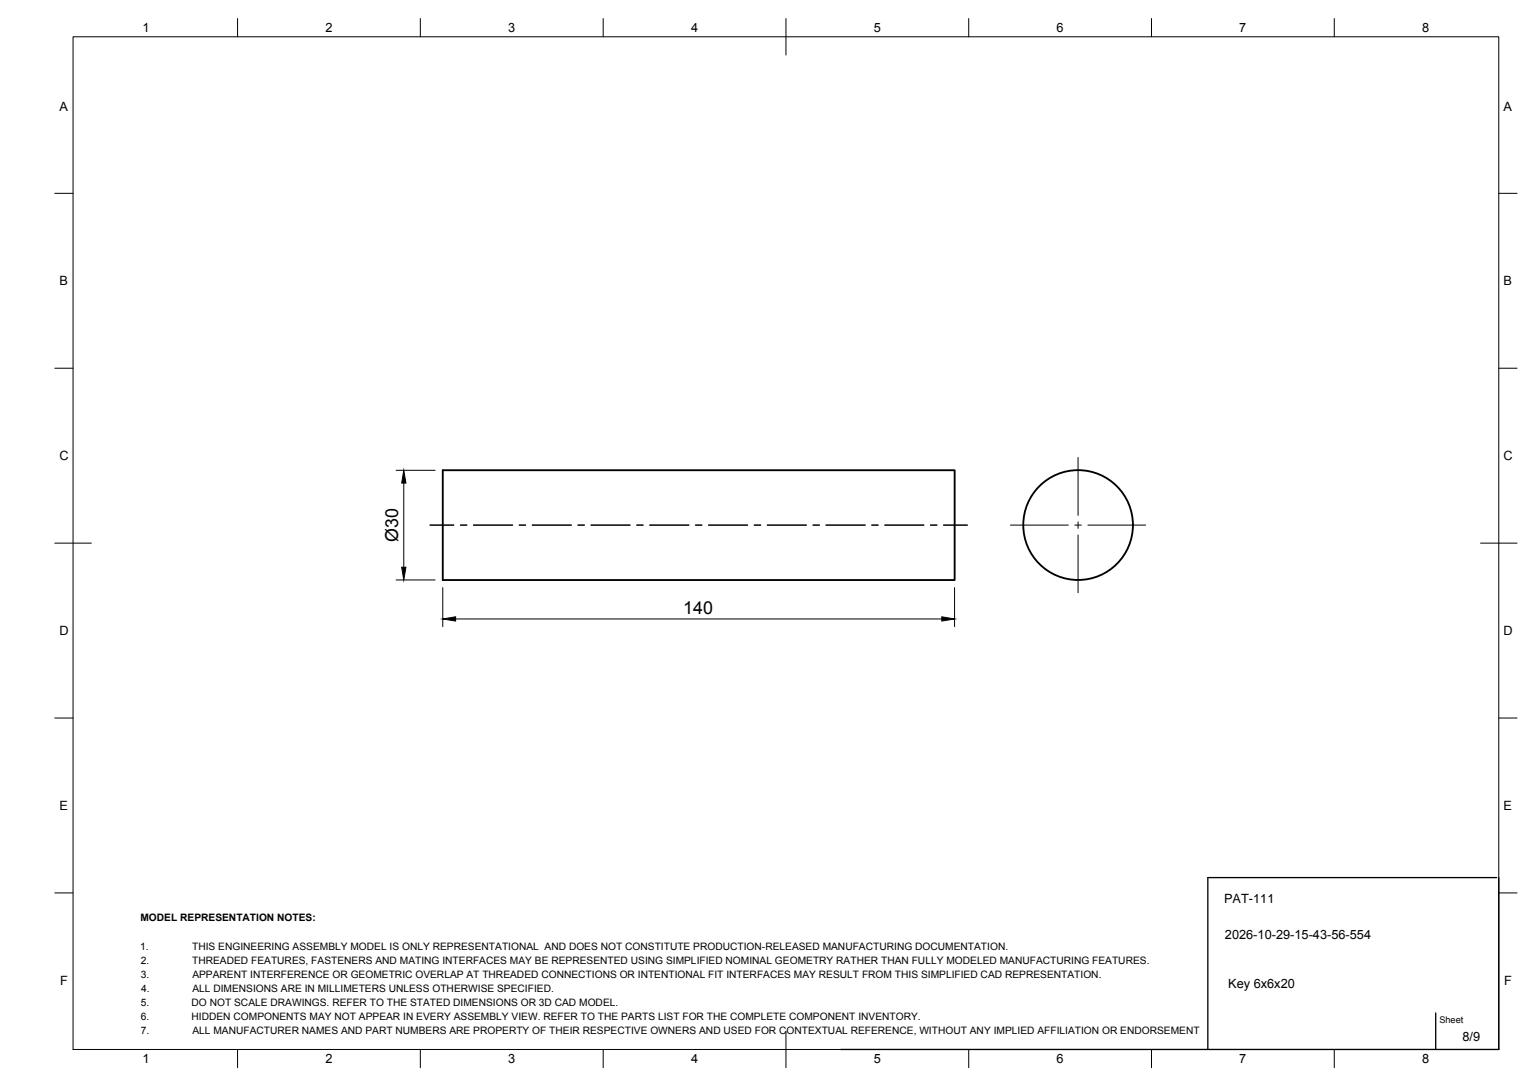
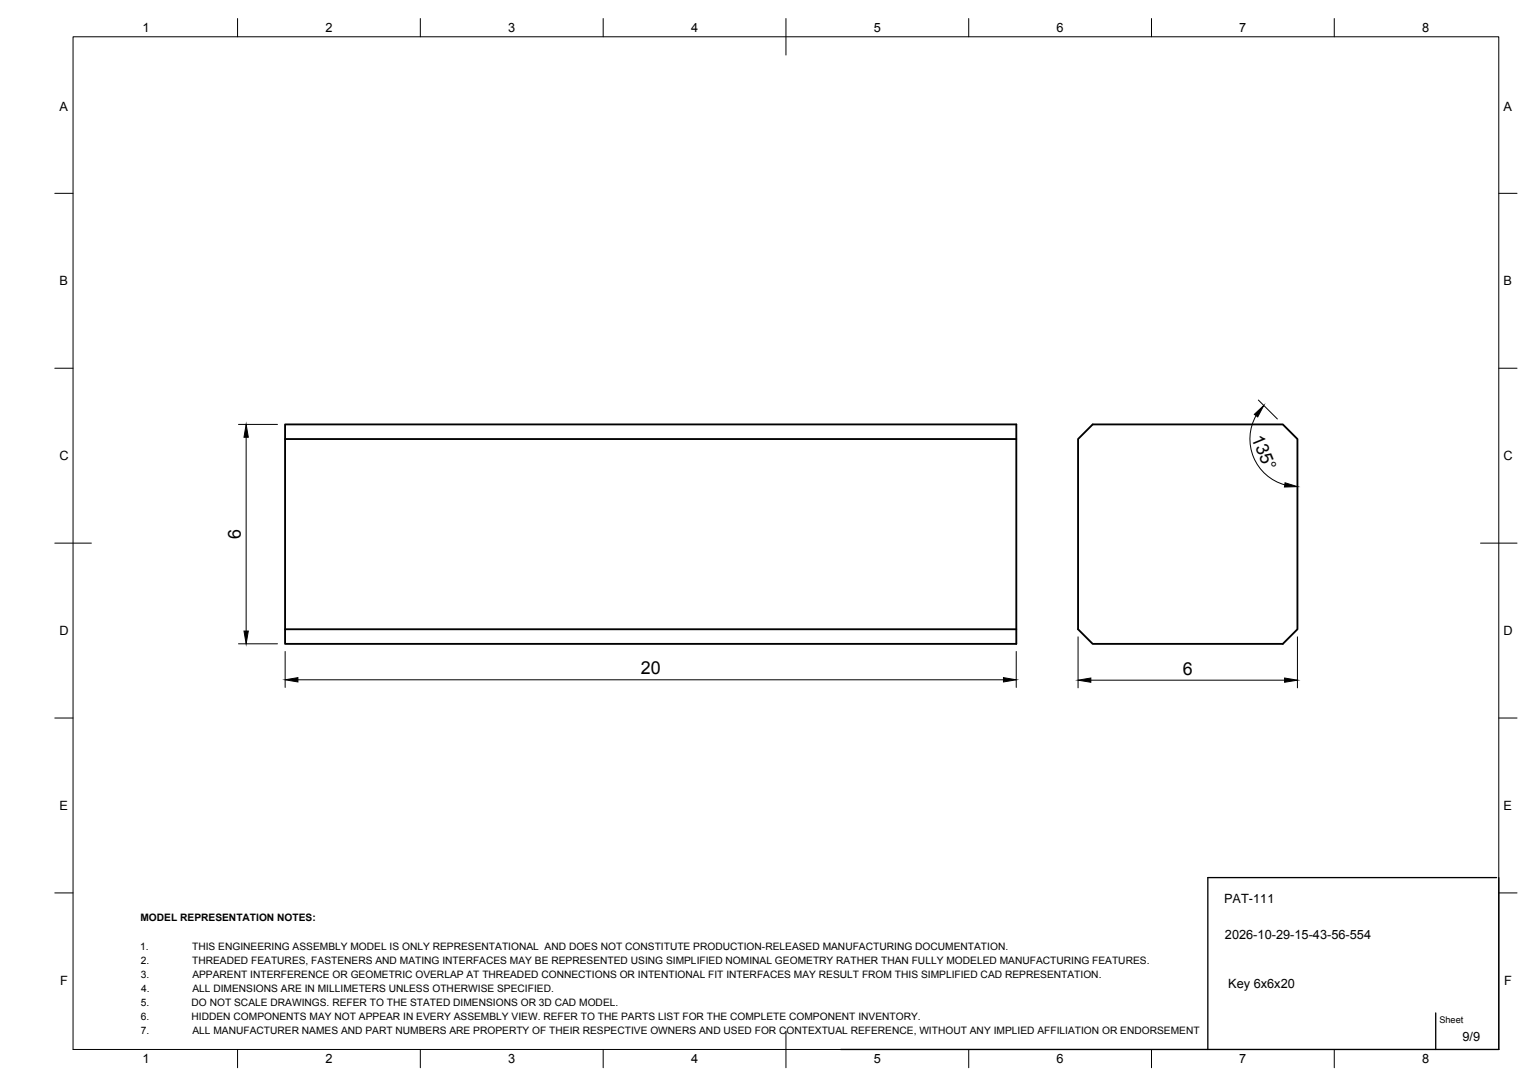
ISO-10303-21;
HEADER;
/* Generated by software containing ST-Developer
 * from STEP Tools, Inc. (www.steptools.com) 
 */

FILE_DESCRIPTION(
/* description */ ('Grid plate located blocks and clamp'),
/* implementation_level */ '2;1');

FILE_NAME(
/* name */ 'Key 6x6x20.step',
/* time_stamp */ '2026-10-29T15:43:47-07:00',
/* author */ (''),
/* organization */ (''),
/* preprocessor_version */ 'ST-DEVELOPER v20.2',
/* originating_system */ 'Autodesk Translation Framework v15.17.0.0',
/* authorisation */ '');

FILE_SCHEMA (('AUTOMOTIVE_DESIGN { 1 0 10303 214 3 1 1 }'));
ENDSEC;

DATA;
#10=MECHANICAL_DESIGN_GEOMETRIC_PRESENTATION_REPRESENTATION('',(#167),#5702);
#143=SHAPE_REPRESENTATION_RELATIONSHIP('SRR','None',#5761,#155);
#155=ADVANCED_BREP_SHAPE_REPRESENTATION('',(#181),#5691);
#167=STYLED_ITEM('',(#5897),#181);
#181=MANIFOLD_SOLID_BREP('Body1',#3262);
#498=FACE_OUTER_BOUND('',#733,.T.);
#499=FACE_OUTER_BOUND('',#734,.T.);
#500=FACE_OUTER_BOUND('',#735,.T.);
#501=FACE_OUTER_BOUND('',#736,.T.);
#502=FACE_OUTER_BOUND('',#737,.T.);
#503=FACE_OUTER_BOUND('',#738,.T.);
#504=FACE_OUTER_BOUND('',#739,.T.);
#505=FACE_OUTER_BOUND('',#740,.T.);
#506=FACE_OUTER_BOUND('',#741,.T.);
#507=FACE_OUTER_BOUND('',#742,.T.);
#733=EDGE_LOOP('',(#2354,#2355,#2356,#2357,#2358,#2359,#2360,#2361));
#734=EDGE_LOOP('',(#2362,#2363,#2364,#2365));
#735=EDGE_LOOP('',(#2366,#2367,#2368,#2369));
#736=EDGE_LOOP('',(#2370,#2371,#2372,#2373));
#737=EDGE_LOOP('',(#2374,#2375,#2376,#2377));
#738=EDGE_LOOP('',(#2378,#2379,#2380,#2381,#2382,#2383,#2384,#2385));
#739=EDGE_LOOP('',(#2386,#2387,#2388,#2389));
#740=EDGE_LOOP('',(#2390,#2391,#2392,#2393));
#741=EDGE_LOOP('',(#2394,#2395,#2396,#2397));
#742=EDGE_LOOP('',(#2398,#2399,#2400,#2401));
#960=LINE('',#4974,#1233);
#961=LINE('',#4976,#1234);
#962=LINE('',#4978,#1235);
#963=LINE('',#4980,#1236);
#964=LINE('',#4982,#1237);
#965=LINE('',#4984,#1238);
#966=LINE('',#4986,#1239);
#967=LINE('',#4987,#1240);
#968=LINE('',#4990,#1241);
#969=LINE('',#4992,#1242);
#970=LINE('',#4993,#1243);
#971=LINE('',#4996,#1244);
#972=LINE('',#4997,#1245);
#973=LINE('',#5000,#1246);
#974=LINE('',#5001,#1247);
#975=LINE('',#5004,#1248);
#976=LINE('',#5005,#1249);
#977=LINE('',#5009,#1250);
#978=LINE('',#5010,#1251);
#979=LINE('',#5012,#1252);
#980=LINE('',#5013,#1253);
#981=LINE('',#5015,#1254);
#982=LINE('',#5017,#1255);
#983=LINE('',#5019,#1256);
#1233=VECTOR('',#4014,1.);
#1234=VECTOR('',#4015,1.);
#1235=VECTOR('',#4016,1.);
#1236=VECTOR('',#4017,1.);
#1237=VECTOR('',#4018,1.);
#1238=VECTOR('',#4019,1.);
#1239=VECTOR('',#4020,1.);
#1240=VECTOR('',#4021,1.);
#1241=VECTOR('',#4024,1.);
#1242=VECTOR('',#4025,1.);
#1243=VECTOR('',#4026,1.);
#1244=VECTOR('',#4029,1.);
#1245=VECTOR('',#4030,1.);
#1246=VECTOR('',#4033,1.);
#1247=VECTOR('',#4034,1.);
#1248=VECTOR('',#4037,1.);
#1249=VECTOR('',#4038,1.);
#1250=VECTOR('',#4041,1.);
#1251=VECTOR('',#4042,1.);
#1252=VECTOR('',#4043,1.);
#1253=VECTOR('',#4044,1.);
#1254=VECTOR('',#4047,1.);
#1255=VECTOR('',#4050,1.);
#1256=VECTOR('',#4053,1.);
#1519=VERTEX_POINT('',#4972);
#1520=VERTEX_POINT('',#4973);
#1521=VERTEX_POINT('',#4975);
#1522=VERTEX_POINT('',#4977);
#1523=VERTEX_POINT('',#4979);
#1524=VERTEX_POINT('',#4981);
#1525=VERTEX_POINT('',#4983);
#1526=VERTEX_POINT('',#4985);
#1527=VERTEX_POINT('',#4989);
#1528=VERTEX_POINT('',#4991);
#1529=VERTEX_POINT('',#4995);
#1530=VERTEX_POINT('',#4999);
#1531=VERTEX_POINT('',#5003);
#1532=VERTEX_POINT('',#5007);
#1533=VERTEX_POINT('',#5008);
#1534=VERTEX_POINT('',#5011);
#1827=EDGE_CURVE('',#1519,#1520,#960,.T.);
#1828=EDGE_CURVE('',#1521,#1519,#961,.T.);
#1829=EDGE_CURVE('',#1522,#1521,#962,.T.);
#1830=EDGE_CURVE('',#1523,#1522,#963,.T.);
#1831=EDGE_CURVE('',#1524,#1523,#964,.T.);
#1832=EDGE_CURVE('',#1525,#1524,#965,.T.);
#1833=EDGE_CURVE('',#1526,#1525,#966,.T.);
#1834=EDGE_CURVE('',#1520,#1526,#967,.T.);
#1835=EDGE_CURVE('',#1523,#1527,#968,.T.);
#1836=EDGE_CURVE('',#1527,#1528,#969,.T.);
#1837=EDGE_CURVE('',#1528,#1524,#970,.T.);
#1838=EDGE_CURVE('',#1529,#1522,#971,.T.);
#1839=EDGE_CURVE('',#1529,#1527,#972,.T.);
#1840=EDGE_CURVE('',#1521,#1530,#973,.T.);
#1841=EDGE_CURVE('',#1530,#1529,#974,.T.);
#1842=EDGE_CURVE('',#1531,#1519,#975,.T.);
#1843=EDGE_CURVE('',#1531,#1530,#976,.T.);
#1844=EDGE_CURVE('',#1532,#1533,#977,.T.);
#1845=EDGE_CURVE('',#1528,#1532,#978,.T.);
#1846=EDGE_CURVE('',#1534,#1531,#979,.T.);
#1847=EDGE_CURVE('',#1533,#1534,#980,.T.);
#1848=EDGE_CURVE('',#1525,#1532,#981,.T.);
#1849=EDGE_CURVE('',#1520,#1534,#982,.T.);
#1850=EDGE_CURVE('',#1533,#1526,#983,.T.);
#2354=ORIENTED_EDGE('',*,*,#1827,.F.);
#2355=ORIENTED_EDGE('',*,*,#1828,.F.);
#2356=ORIENTED_EDGE('',*,*,#1829,.F.);
#2357=ORIENTED_EDGE('',*,*,#1830,.F.);
#2358=ORIENTED_EDGE('',*,*,#1831,.F.);
#2359=ORIENTED_EDGE('',*,*,#1832,.F.);
#2360=ORIENTED_EDGE('',*,*,#1833,.F.);
#2361=ORIENTED_EDGE('',*,*,#1834,.F.);
#2362=ORIENTED_EDGE('',*,*,#1831,.T.);
#2363=ORIENTED_EDGE('',*,*,#1835,.T.);
#2364=ORIENTED_EDGE('',*,*,#1836,.T.);
#2365=ORIENTED_EDGE('',*,*,#1837,.T.);
#2366=ORIENTED_EDGE('',*,*,#1830,.T.);
#2367=ORIENTED_EDGE('',*,*,#1838,.F.);
#2368=ORIENTED_EDGE('',*,*,#1839,.T.);
#2369=ORIENTED_EDGE('',*,*,#1835,.F.);
#2370=ORIENTED_EDGE('',*,*,#1829,.T.);
#2371=ORIENTED_EDGE('',*,*,#1840,.T.);
#2372=ORIENTED_EDGE('',*,*,#1841,.T.);
#2373=ORIENTED_EDGE('',*,*,#1838,.T.);
#2374=ORIENTED_EDGE('',*,*,#1828,.T.);
#2375=ORIENTED_EDGE('',*,*,#1842,.F.);
#2376=ORIENTED_EDGE('',*,*,#1843,.T.);
#2377=ORIENTED_EDGE('',*,*,#1840,.F.);
#2378=ORIENTED_EDGE('',*,*,#1844,.F.);
#2379=ORIENTED_EDGE('',*,*,#1845,.F.);
#2380=ORIENTED_EDGE('',*,*,#1836,.F.);
#2381=ORIENTED_EDGE('',*,*,#1839,.F.);
#2382=ORIENTED_EDGE('',*,*,#1841,.F.);
#2383=ORIENTED_EDGE('',*,*,#1843,.F.);
#2384=ORIENTED_EDGE('',*,*,#1846,.F.);
#2385=ORIENTED_EDGE('',*,*,#1847,.F.);
#2386=ORIENTED_EDGE('',*,*,#1832,.T.);
#2387=ORIENTED_EDGE('',*,*,#1837,.F.);
#2388=ORIENTED_EDGE('',*,*,#1845,.T.);
#2389=ORIENTED_EDGE('',*,*,#1848,.F.);
#2390=ORIENTED_EDGE('',*,*,#1827,.T.);
#2391=ORIENTED_EDGE('',*,*,#1849,.T.);
#2392=ORIENTED_EDGE('',*,*,#1846,.T.);
#2393=ORIENTED_EDGE('',*,*,#1842,.T.);
#2394=ORIENTED_EDGE('',*,*,#1833,.T.);
#2395=ORIENTED_EDGE('',*,*,#1848,.T.);
#2396=ORIENTED_EDGE('',*,*,#1844,.T.);
#2397=ORIENTED_EDGE('',*,*,#1850,.T.);
#2398=ORIENTED_EDGE('',*,*,#1834,.T.);
#2399=ORIENTED_EDGE('',*,*,#1850,.F.);
#2400=ORIENTED_EDGE('',*,*,#1847,.T.);
#2401=ORIENTED_EDGE('',*,*,#1849,.F.);
#2980=PLANE('',#3504);
#2981=PLANE('',#3505);
#2982=PLANE('',#3506);
#2983=PLANE('',#3507);
#2984=PLANE('',#3508);
#2985=PLANE('',#3509);
#2986=PLANE('',#3510);
#2987=PLANE('',#3511);
#2988=PLANE('',#3512);
#2989=PLANE('',#3513);
#3119=ADVANCED_FACE('',(#498),#2980,.F.);
#3120=ADVANCED_FACE('',(#499),#2981,.T.);
#3121=ADVANCED_FACE('',(#500),#2982,.T.);
#3122=ADVANCED_FACE('',(#501),#2983,.T.);
#3123=ADVANCED_FACE('',(#502),#2984,.T.);
#3124=ADVANCED_FACE('',(#503),#2985,.T.);
#3125=ADVANCED_FACE('',(#504),#2986,.F.);
#3126=ADVANCED_FACE('',(#505),#2987,.T.);
#3127=ADVANCED_FACE('',(#506),#2988,.T.);
#3128=ADVANCED_FACE('',(#507),#2989,.T.);
#3262=CLOSED_SHELL('',(#3119,#3120,#3121,#3122,#3123,#3124,#3125,#3126,
#3127,#3128));
#3503=AXIS2_PLACEMENT_3D('',#4970,#4010,#4011);
#3504=AXIS2_PLACEMENT_3D('',#4971,#4012,#4013);
#3505=AXIS2_PLACEMENT_3D('',#4988,#4022,#4023);
#3506=AXIS2_PLACEMENT_3D('',#4994,#4027,#4028);
#3507=AXIS2_PLACEMENT_3D('',#4998,#4031,#4032);
#3508=AXIS2_PLACEMENT_3D('',#5002,#4035,#4036);
#3509=AXIS2_PLACEMENT_3D('',#5006,#4039,#4040);
#3510=AXIS2_PLACEMENT_3D('',#5014,#4045,#4046);
#3511=AXIS2_PLACEMENT_3D('',#5016,#4048,#4049);
#3512=AXIS2_PLACEMENT_3D('',#5018,#4051,#4052);
#3513=AXIS2_PLACEMENT_3D('',#5020,#4054,#4055);
#4010=DIRECTION('axis',(0.,0.,1.));
#4011=DIRECTION('refdir',(1.,0.,0.));
#4012=DIRECTION('center_axis',(1.,0.,0.));
#4013=DIRECTION('ref_axis',(0.,0.,-1.));
#4014=DIRECTION('',(0.,-0.707106781186547,-0.707106781186548));
#4015=DIRECTION('',(0.,-1.,0.));
#4016=DIRECTION('',(0.,-0.707106781186547,0.707106781186548));
#4017=DIRECTION('',(0.,0.,1.));
#4018=DIRECTION('',(0.,0.707106781186547,0.707106781186548));
#4019=DIRECTION('',(0.,1.,0.));
#4020=DIRECTION('',(0.,0.707106781186547,-0.707106781186548));
#4021=DIRECTION('',(0.,0.,-1.));
#4022=DIRECTION('center_axis',(0.,0.707106781186548,-0.707106781186547));
#4023=DIRECTION('ref_axis',(-1.,0.,0.));
#4024=DIRECTION('',(1.,0.,0.));
#4025=DIRECTION('',(0.,-0.707106781186547,-0.707106781186548));
#4026=DIRECTION('',(-1.,0.,0.));
#4027=DIRECTION('center_axis',(0.,1.,0.));
#4028=DIRECTION('ref_axis',(-1.,0.,0.));
#4029=DIRECTION('',(-1.,0.,0.));
#4030=DIRECTION('',(0.,0.,-1.));
#4031=DIRECTION('center_axis',(0.,0.707106781186548,0.707106781186547));
#4032=DIRECTION('ref_axis',(1.,0.,0.));
#4033=DIRECTION('',(1.,0.,0.));
#4034=DIRECTION('',(0.,0.707106781186547,-0.707106781186548));
#4035=DIRECTION('center_axis',(0.,0.,1.));
#4036=DIRECTION('ref_axis',(1.,0.,0.));
#4037=DIRECTION('',(-1.,0.,0.));
#4038=DIRECTION('',(0.,1.,0.));
#4039=DIRECTION('center_axis',(1.,0.,0.));
#4040=DIRECTION('ref_axis',(0.,0.,-1.));
#4041=DIRECTION('',(0.,-0.707106781186547,0.707106781186548));
#4042=DIRECTION('',(0.,-1.,0.));
#4043=DIRECTION('',(0.,0.707106781186547,0.707106781186548));
#4044=DIRECTION('',(0.,0.,1.));
#4045=DIRECTION('center_axis',(0.,0.,1.));
#4046=DIRECTION('ref_axis',(1.,0.,0.));
#4047=DIRECTION('',(1.,0.,0.));
#4048=DIRECTION('center_axis',(0.,-0.707106781186548,0.707106781186547));
#4049=DIRECTION('ref_axis',(1.,0.,0.));
#4050=DIRECTION('',(1.,0.,0.));
#4051=DIRECTION('center_axis',(0.,-0.707106781186548,-0.707106781186547));
#4052=DIRECTION('ref_axis',(-1.,0.,0.));
#4053=DIRECTION('',(-1.,0.,0.));
#4054=DIRECTION('center_axis',(0.,-1.,0.));
#4055=DIRECTION('ref_axis',(1.,0.,0.));
#4970=CARTESIAN_POINT('',(0.,0.,0.));
#4971=CARTESIAN_POINT('Origin',(-1.,0.,0.35));
#4972=CARTESIAN_POINT('',(-1.,-0.26,0.6));
#4973=CARTESIAN_POINT('',(-1.,-0.3,0.56));
#4974=CARTESIAN_POINT('',(-1.,-0.2675,0.5925));
#4975=CARTESIAN_POINT('',(-1.,0.26,0.6));
#4976=CARTESIAN_POINT('',(-1.,0.,0.6));
#4977=CARTESIAN_POINT('',(-1.,0.3,0.56));
#4978=CARTESIAN_POINT('',(-1.,0.2675,0.5925));
#4979=CARTESIAN_POINT('',(-1.,0.3,0.04));
#4980=CARTESIAN_POINT('',(-1.,0.3,0.175));
#4981=CARTESIAN_POINT('',(-1.,0.26,0.));
#4982=CARTESIAN_POINT('',(-1.,0.2925,0.0325));
#4983=CARTESIAN_POINT('',(-1.,-0.26,0.));
#4984=CARTESIAN_POINT('',(-1.,0.,0.));
#4985=CARTESIAN_POINT('',(-1.,-0.3,0.04));
#4986=CARTESIAN_POINT('',(-1.,-0.2925,0.0325));
#4987=CARTESIAN_POINT('',(-1.,-0.3,0.175));
#4988=CARTESIAN_POINT('Origin',(0.75,0.28,0.02));
#4989=CARTESIAN_POINT('',(1.,0.3,0.04));
#4990=CARTESIAN_POINT('',(0.75,0.3,0.04));
#4991=CARTESIAN_POINT('',(1.,0.26,0.));
#4992=CARTESIAN_POINT('',(1.,0.2925,0.0325));
#4993=CARTESIAN_POINT('',(0.75,0.26,0.));
#4994=CARTESIAN_POINT('Origin',(1.5,0.3,0.));
#4995=CARTESIAN_POINT('',(1.,0.3,0.56));
#4996=CARTESIAN_POINT('',(0.75,0.3,0.56));
#4997=CARTESIAN_POINT('',(1.,0.3,0.175));
#4998=CARTESIAN_POINT('Origin',(0.75,0.28,0.58));
#4999=CARTESIAN_POINT('',(1.,0.26,0.6));
#5000=CARTESIAN_POINT('',(0.75,0.26,0.6));
#5001=CARTESIAN_POINT('',(1.,0.2675,0.5925));
#5002=CARTESIAN_POINT('Origin',(0.,0.,0.6));
#5003=CARTESIAN_POINT('',(1.,-0.26,0.6));
#5004=CARTESIAN_POINT('',(-0.75,-0.26,0.6));
#5005=CARTESIAN_POINT('',(1.,0.,0.6));
#5006=CARTESIAN_POINT('Origin',(1.,0.,0.35));
#5007=CARTESIAN_POINT('',(1.,-0.26,0.));
#5008=CARTESIAN_POINT('',(1.,-0.3,0.04));
#5009=CARTESIAN_POINT('',(1.,-0.2925,0.0325));
#5010=CARTESIAN_POINT('',(1.,0.,0.));
#5011=CARTESIAN_POINT('',(1.,-0.3,0.56));
#5012=CARTESIAN_POINT('',(1.,-0.2675,0.5925));
#5013=CARTESIAN_POINT('',(1.,-0.3,0.175));
#5014=CARTESIAN_POINT('Origin',(0.,0.,0.));
#5015=CARTESIAN_POINT('',(-0.75,-0.26,0.));
#5016=CARTESIAN_POINT('Origin',(-0.75,-0.28,0.58));
#5017=CARTESIAN_POINT('',(-0.75,-0.3,0.56));
#5018=CARTESIAN_POINT('Origin',(-0.75,-0.28,0.02));
#5019=CARTESIAN_POINT('',(-0.75,-0.3,0.04));
#5020=CARTESIAN_POINT('Origin',(-1.5,-0.3,0.));
#5677=UNCERTAINTY_MEASURE_WITH_UNIT(LENGTH_MEASURE(0.001),#5703,
'DISTANCE_ACCURACY_VALUE',
'Maximum model space distance between geometric entities at asserted c
onnectivities');
#5688=UNCERTAINTY_MEASURE_WITH_UNIT(LENGTH_MEASURE(0.001),#5703,
'DISTANCE_ACCURACY_VALUE',
'Maximum model space distance between geometric entities at asserted c
onnectivities');
#5691=(
GEOMETRIC_REPRESENTATION_CONTEXT(3)
GLOBAL_UNCERTAINTY_ASSIGNED_CONTEXT((#5677))
GLOBAL_UNIT_ASSIGNED_CONTEXT((#5703,#5705,#5706))
REPRESENTATION_CONTEXT('','3D')
);
#5702=(
GEOMETRIC_REPRESENTATION_CONTEXT(3)
GLOBAL_UNCERTAINTY_ASSIGNED_CONTEXT((#5688))
GLOBAL_UNIT_ASSIGNED_CONTEXT((#5703,#5705,#5706))
REPRESENTATION_CONTEXT('','3D')
);
#5703=(
LENGTH_UNIT()
NAMED_UNIT(*)
SI_UNIT(.CENTI.,.METRE.)
);
#5705=(
NAMED_UNIT(*)
PLANE_ANGLE_UNIT()
SI_UNIT($,.RADIAN.)
);
#5706=(
NAMED_UNIT(*)
SI_UNIT($,.STERADIAN.)
SOLID_ANGLE_UNIT()
);
#5709=SHAPE_DEFINITION_REPRESENTATION(#5722,#5761);
#5722=PRODUCT_DEFINITION_SHAPE('',$,#5775);
#5761=SHAPE_REPRESENTATION('',(#3503),#5691);
#5772=PRODUCT_DEFINITION_CONTEXT('part definition',#5813,'design');
#5775=PRODUCT_DEFINITION('Key 6x6x20','Key 6x6x20',#5788,#5772);
#5788=PRODUCT_DEFINITION_FORMATION('',$,#5817);
#5813=APPLICATION_CONTEXT(
'Core Data for Automotive Mechanical Design Process');
#5814=PRODUCT_CONTEXT('part definition',#5813,'mechanical');
#5817=PRODUCT('Key 6x6x20','Key 6x6x20','Key 6x6x20',(#5814));
#5891=COLOUR_RGB('Grey',0.48,0.52,0.57);
#5892=FILL_AREA_STYLE_COLOUR('',#5891);
#5893=FILL_AREA_STYLE('',(#5892));
#5894=SURFACE_STYLE_FILL_AREA(#5893);
#5895=SURFACE_SIDE_STYLE('',(#5894));
#5896=SURFACE_STYLE_USAGE(.BOTH.,#5895);
#5897=PRESENTATION_STYLE_ASSIGNMENT((#5896));
ENDSEC;
END-ISO-10303-21;
